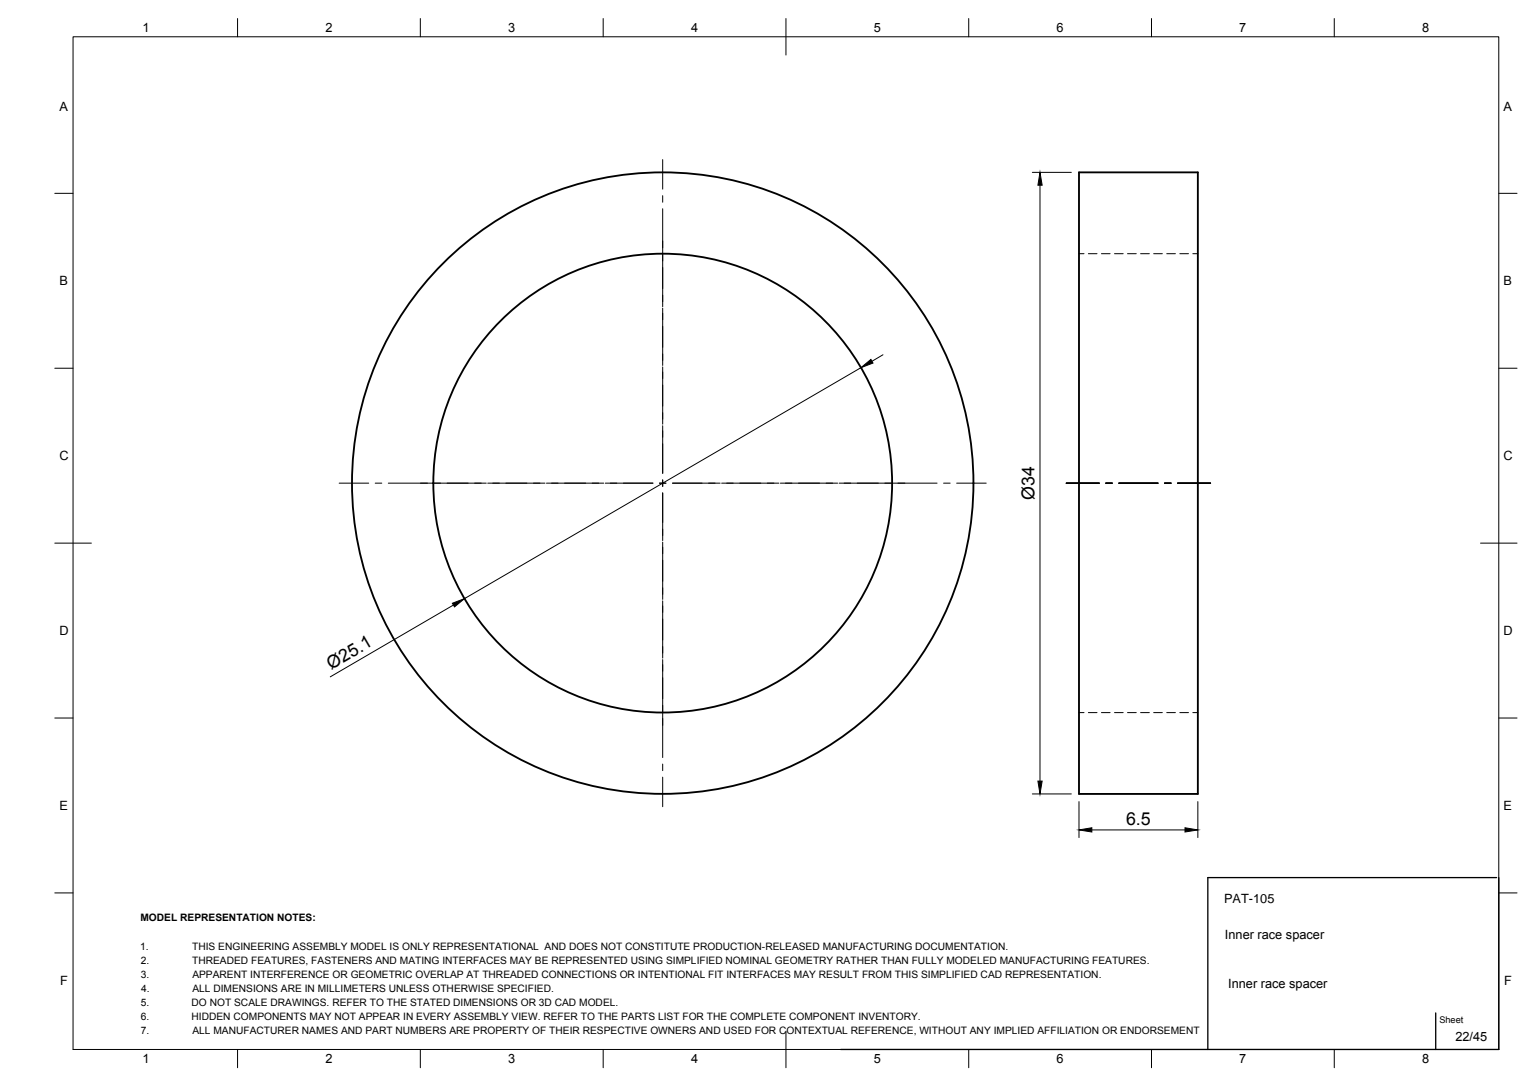
ISO-10303-21;
HEADER;
/* Generated by software containing ST-Developer
 * from STEP Tools, Inc. (www.steptools.com) 
 */

FILE_DESCRIPTION(
/* description */ ('Torque wrench calibration arm'),
/* implementation_level */ '2;1');

FILE_NAME(
/* name */ 'Inner race spacer.step',
/* time_stamp */ '2026-10-28T03:24:52-07:00',
/* author */ (''),
/* organization */ (''),
/* preprocessor_version */ 'ST-DEVELOPER v20.2',
/* originating_system */ 'Autodesk Translation Framework v15.17.0.0',
/* authorisation */ '');

FILE_SCHEMA (('AUTOMOTIVE_DESIGN { 1 0 10303 214 3 1 1 }'));
ENDSEC;

DATA;
#10=MECHANICAL_DESIGN_GEOMETRIC_PRESENTATION_REPRESENTATION('',(#450),#12783);
#367=SHAPE_REPRESENTATION_RELATIONSHIP('SRR','None',#12950,#404);
#404=ADVANCED_BREP_SHAPE_REPRESENTATION('',(#502),#12759);
#450=STYLED_ITEM('',(#13212),#502);
#502=MANIFOLD_SOLID_BREP('Body1',#6521);
#598=FACE_BOUND('',#1545,.T.);
#599=FACE_BOUND('',#1547,.T.);
#764=PLANE('',#7410);
#765=PLANE('',#7411);
#1080=FACE_OUTER_BOUND('',#1542,.T.);
#1081=FACE_OUTER_BOUND('',#1543,.T.);
#1082=FACE_OUTER_BOUND('',#1544,.T.);
#1083=FACE_OUTER_BOUND('',#1546,.T.);
#1542=EDGE_LOOP('',(#5215,#5216,#5217,#5218));
#1543=EDGE_LOOP('',(#5219,#5220,#5221,#5222));
#1544=EDGE_LOOP('',(#5223));
#1545=EDGE_LOOP('',(#5224));
#1546=EDGE_LOOP('',(#5225));
#1547=EDGE_LOOP('',(#5226));
#2007=LINE('',#11286,#2422);
#2008=LINE('',#11292,#2423);
#2422=VECTOR('',#8923,1.255);
#2423=VECTOR('',#8930,1.7);
#2809=CIRCLE('',#7405,1.255);
#2810=CIRCLE('',#7406,1.255);
#2811=CIRCLE('',#7408,1.7);
#2812=CIRCLE('',#7409,1.7);
#3267=VERTEX_POINT('',#11283);
#3268=VERTEX_POINT('',#11285);
#3269=VERTEX_POINT('',#11289);
#3270=VERTEX_POINT('',#11291);
#3965=EDGE_CURVE('',#3267,#3267,#2809,.T.);
#3966=EDGE_CURVE('',#3267,#3268,#2007,.T.);
#3967=EDGE_CURVE('',#3268,#3268,#2810,.T.);
#3968=EDGE_CURVE('',#3269,#3269,#2811,.T.);
#3969=EDGE_CURVE('',#3269,#3270,#2008,.T.);
#3970=EDGE_CURVE('',#3270,#3270,#2812,.T.);
#5215=ORIENTED_EDGE('',*,*,#3965,.F.);
#5216=ORIENTED_EDGE('',*,*,#3966,.T.);
#5217=ORIENTED_EDGE('',*,*,#3967,.T.);
#5218=ORIENTED_EDGE('',*,*,#3966,.F.);
#5219=ORIENTED_EDGE('',*,*,#3968,.F.);
#5220=ORIENTED_EDGE('',*,*,#3969,.T.);
#5221=ORIENTED_EDGE('',*,*,#3970,.T.);
#5222=ORIENTED_EDGE('',*,*,#3969,.F.);
#5223=ORIENTED_EDGE('',*,*,#3968,.T.);
#5224=ORIENTED_EDGE('',*,*,#3965,.T.);
#5225=ORIENTED_EDGE('',*,*,#3970,.F.);
#5226=ORIENTED_EDGE('',*,*,#3967,.F.);
#6048=CYLINDRICAL_SURFACE('',#7404,1.255);
#6049=CYLINDRICAL_SURFACE('',#7407,1.7);
#6305=ADVANCED_FACE('',(#1080),#6048,.F.);
#6306=ADVANCED_FACE('',(#1081),#6049,.T.);
#6307=ADVANCED_FACE('',(#1082,#598),#764,.T.);
#6308=ADVANCED_FACE('',(#1083,#599),#765,.F.);
#6521=CLOSED_SHELL('',(#6305,#6306,#6307,#6308));
#7403=AXIS2_PLACEMENT_3D('',#11281,#8917,#8918);
#7404=AXIS2_PLACEMENT_3D('',#11282,#8919,#8920);
#7405=AXIS2_PLACEMENT_3D('',#11284,#8921,#8922);
#7406=AXIS2_PLACEMENT_3D('',#11287,#8924,#8925);
#7407=AXIS2_PLACEMENT_3D('',#11288,#8926,#8927);
#7408=AXIS2_PLACEMENT_3D('',#11290,#8928,#8929);
#7409=AXIS2_PLACEMENT_3D('',#11293,#8931,#8932);
#7410=AXIS2_PLACEMENT_3D('',#11294,#8933,#8934);
#7411=AXIS2_PLACEMENT_3D('',#11295,#8935,#8936);
#8917=DIRECTION('axis',(0.,0.,1.));
#8918=DIRECTION('refdir',(1.,0.,0.));
#8919=DIRECTION('center_axis',(0.,1.,0.));
#8920=DIRECTION('ref_axis',(1.,0.,0.));
#8921=DIRECTION('center_axis',(0.,-1.,0.));
#8922=DIRECTION('ref_axis',(1.,0.,0.));
#8923=DIRECTION('',(0.,-1.,0.));
#8924=DIRECTION('center_axis',(0.,-1.,0.));
#8925=DIRECTION('ref_axis',(1.,0.,0.));
#8926=DIRECTION('center_axis',(0.,1.,0.));
#8927=DIRECTION('ref_axis',(1.,0.,0.));
#8928=DIRECTION('center_axis',(0.,1.,0.));
#8929=DIRECTION('ref_axis',(1.,0.,0.));
#8930=DIRECTION('',(0.,-1.,0.));
#8931=DIRECTION('center_axis',(0.,1.,0.));
#8932=DIRECTION('ref_axis',(1.,0.,0.));
#8933=DIRECTION('center_axis',(0.,1.,0.));
#8934=DIRECTION('ref_axis',(1.,0.,0.));
#8935=DIRECTION('center_axis',(0.,1.,0.));
#8936=DIRECTION('ref_axis',(1.,0.,0.));
#11281=CARTESIAN_POINT('',(0.,0.,0.));
#11282=CARTESIAN_POINT('Origin',(0.,5.75,8.));
#11283=CARTESIAN_POINT('',(-1.255,6.4,8.));
#11284=CARTESIAN_POINT('Origin',(0.,6.4,8.));
#11285=CARTESIAN_POINT('',(-1.255,5.75,8.));
#11286=CARTESIAN_POINT('',(-1.255,5.75,8.));
#11287=CARTESIAN_POINT('Origin',(0.,5.75,8.));
#11288=CARTESIAN_POINT('Origin',(0.,5.75,8.));
#11289=CARTESIAN_POINT('',(-1.7,6.4,8.));
#11290=CARTESIAN_POINT('Origin',(0.,6.4,8.));
#11291=CARTESIAN_POINT('',(-1.7,5.75,8.));
#11292=CARTESIAN_POINT('',(-1.7,5.75,8.));
#11293=CARTESIAN_POINT('Origin',(0.,5.75,8.));
#11294=CARTESIAN_POINT('Origin',(0.,6.4,8.));
#11295=CARTESIAN_POINT('Origin',(0.,5.75,8.));
#12715=UNCERTAINTY_MEASURE_WITH_UNIT(LENGTH_MEASURE(0.001),#12784,
'DISTANCE_ACCURACY_VALUE',
'Maximum model space distance between geometric entities at asserted c
onnectivities');
#12739=UNCERTAINTY_MEASURE_WITH_UNIT(LENGTH_MEASURE(0.001),#12784,
'DISTANCE_ACCURACY_VALUE',
'Maximum model space distance between geometric entities at asserted c
onnectivities');
#12759=(
GEOMETRIC_REPRESENTATION_CONTEXT(3)
GLOBAL_UNCERTAINTY_ASSIGNED_CONTEXT((#12715))
GLOBAL_UNIT_ASSIGNED_CONTEXT((#12784,#12786,#12787))
REPRESENTATION_CONTEXT('','3D')
);
#12783=(
GEOMETRIC_REPRESENTATION_CONTEXT(3)
GLOBAL_UNCERTAINTY_ASSIGNED_CONTEXT((#12739))
GLOBAL_UNIT_ASSIGNED_CONTEXT((#12784,#12786,#12787))
REPRESENTATION_CONTEXT('','3D')
);
#12784=(
LENGTH_UNIT()
NAMED_UNIT(*)
SI_UNIT(.CENTI.,.METRE.)
);
#12786=(
NAMED_UNIT(*)
PLANE_ANGLE_UNIT()
SI_UNIT($,.RADIAN.)
);
#12787=(
NAMED_UNIT(*)
SI_UNIT($,.STERADIAN.)
SOLID_ANGLE_UNIT()
);
#12807=SHAPE_DEFINITION_REPRESENTATION(#12876,#12950);
#12876=PRODUCT_DEFINITION_SHAPE('',$,#12994);
#12950=SHAPE_REPRESENTATION('',(#7403),#12759);
#12974=PRODUCT_DEFINITION_CONTEXT('part definition',#13105,'design');
#12994=PRODUCT_DEFINITION('Inner race spacer','Inner race spacer',#13037,
#12974);
#13037=PRODUCT_DEFINITION_FORMATION('',$,#13126);
#13105=APPLICATION_CONTEXT(
'Core Data for Automotive Mechanical Design Process');
#13106=PRODUCT_CONTEXT('part definition',#13105,'mechanical');
#13126=PRODUCT('Inner race spacer','Inner race spacer',
'Inner race spacer',(#13106));
#13206=COLOUR_RGB('Grey',0.48,0.52,0.57);
#13207=FILL_AREA_STYLE_COLOUR('',#13206);
#13208=FILL_AREA_STYLE('',(#13207));
#13209=SURFACE_STYLE_FILL_AREA(#13208);
#13210=SURFACE_SIDE_STYLE('',(#13209));
#13211=SURFACE_STYLE_USAGE(.BOTH.,#13210);
#13212=PRESENTATION_STYLE_ASSIGNMENT((#13211));
ENDSEC;
END-ISO-10303-21;
